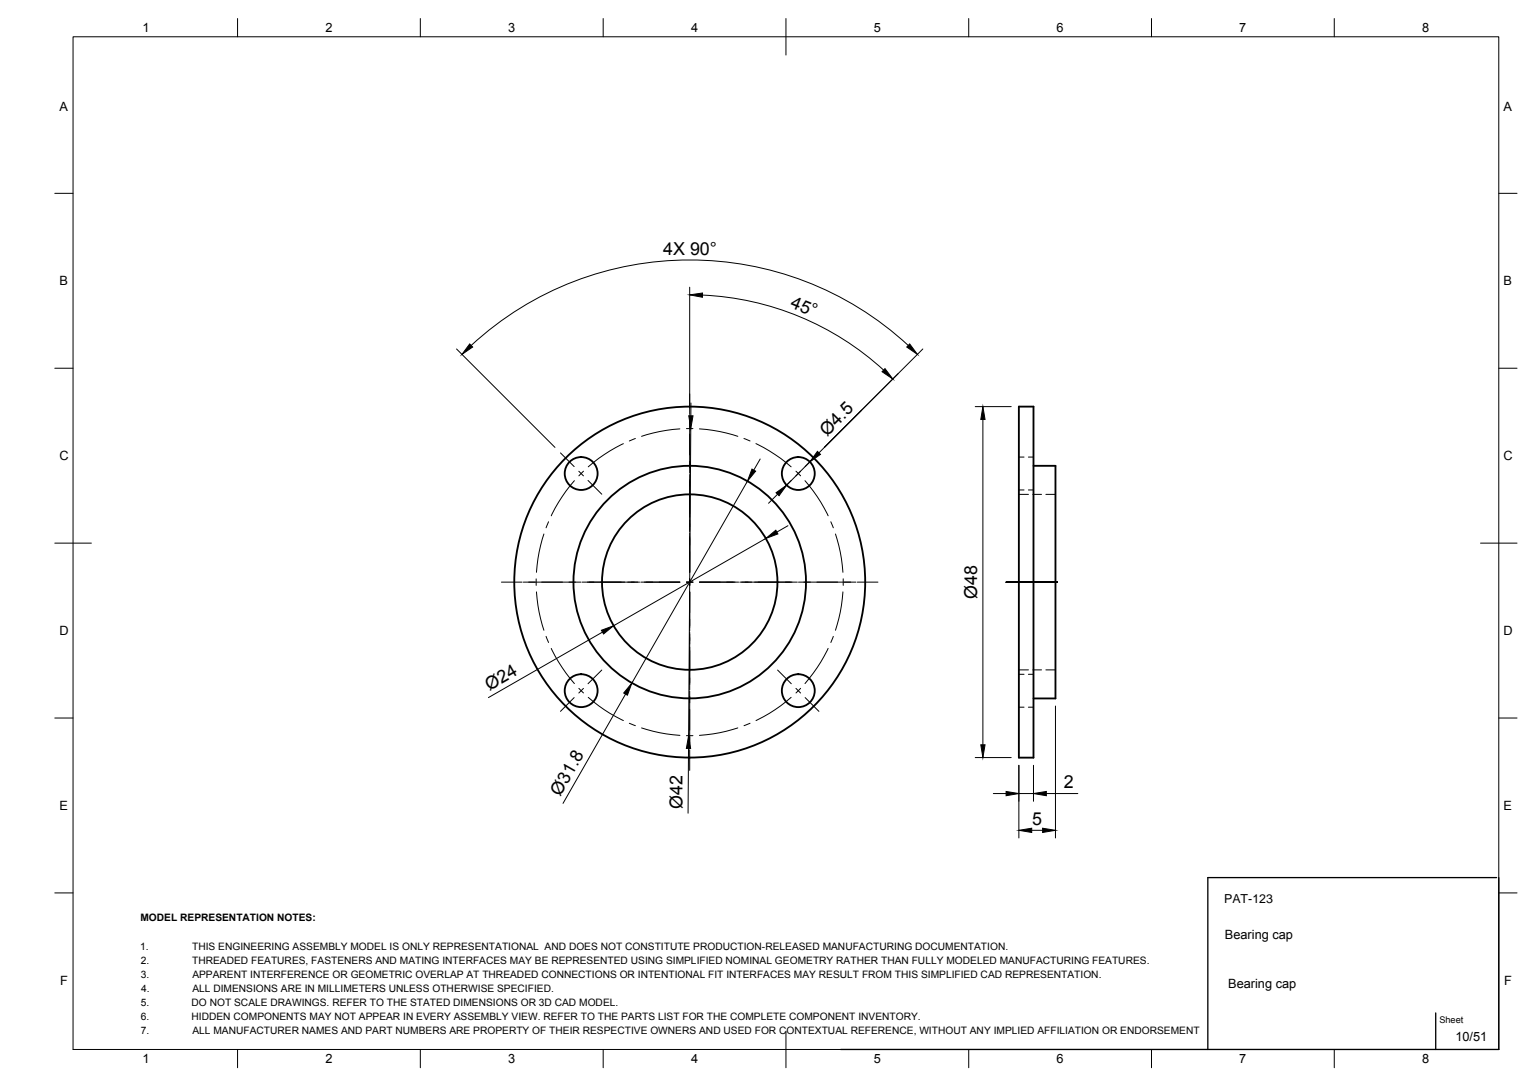
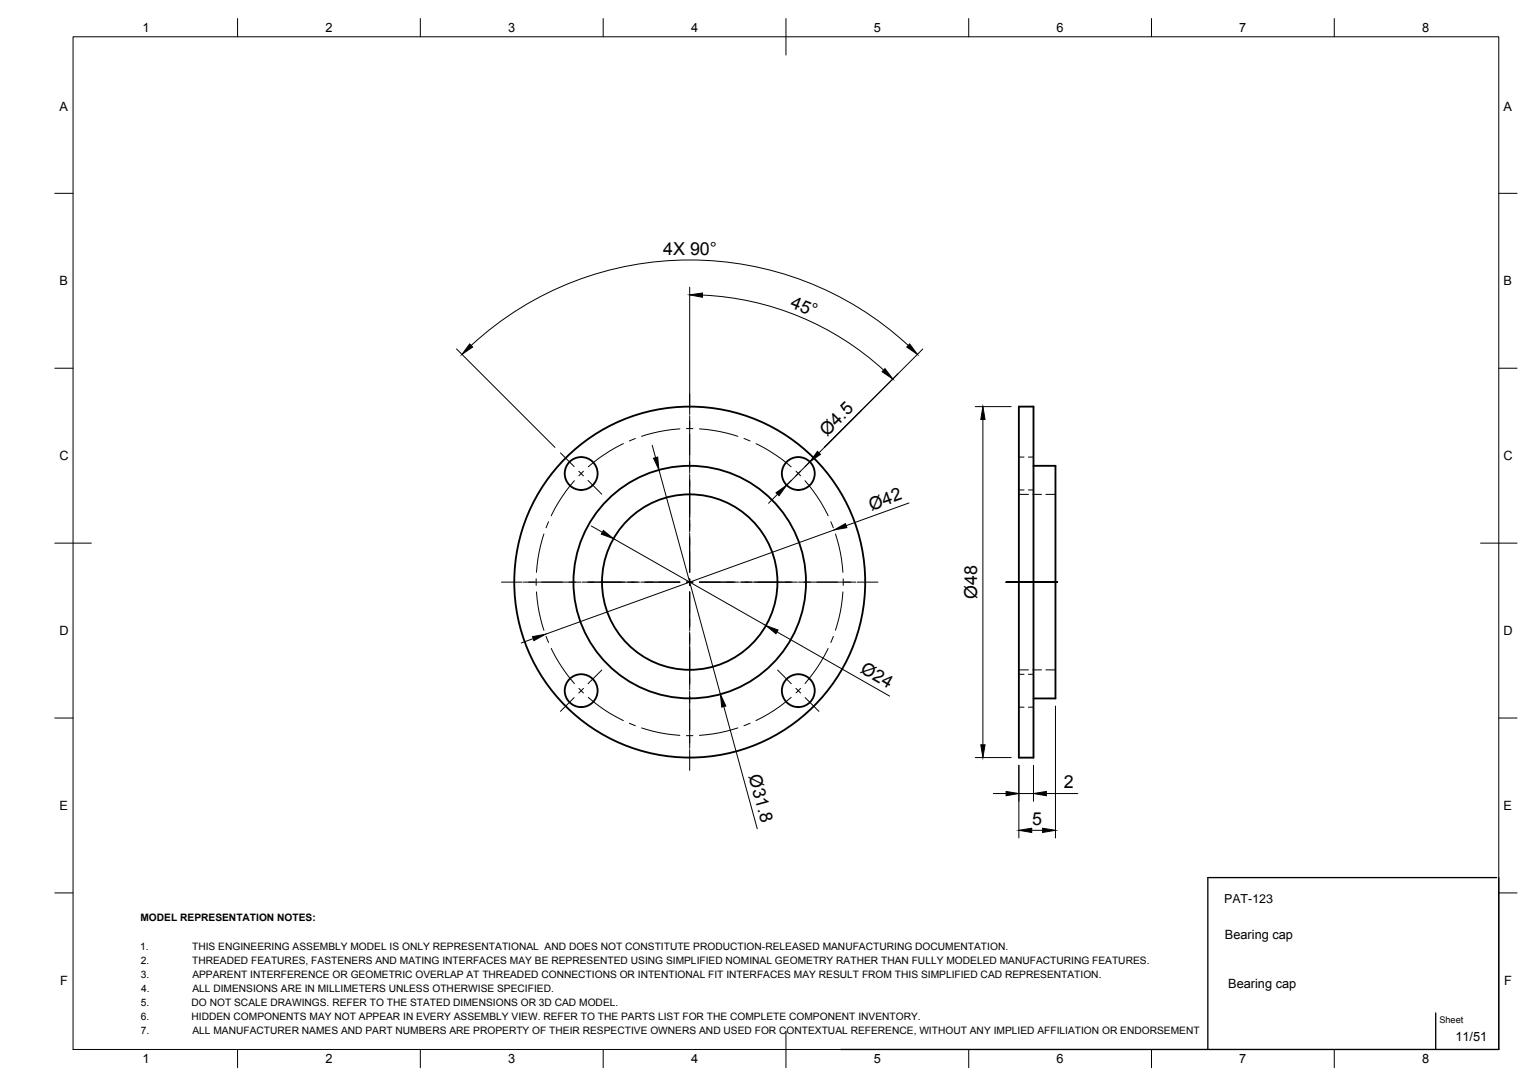
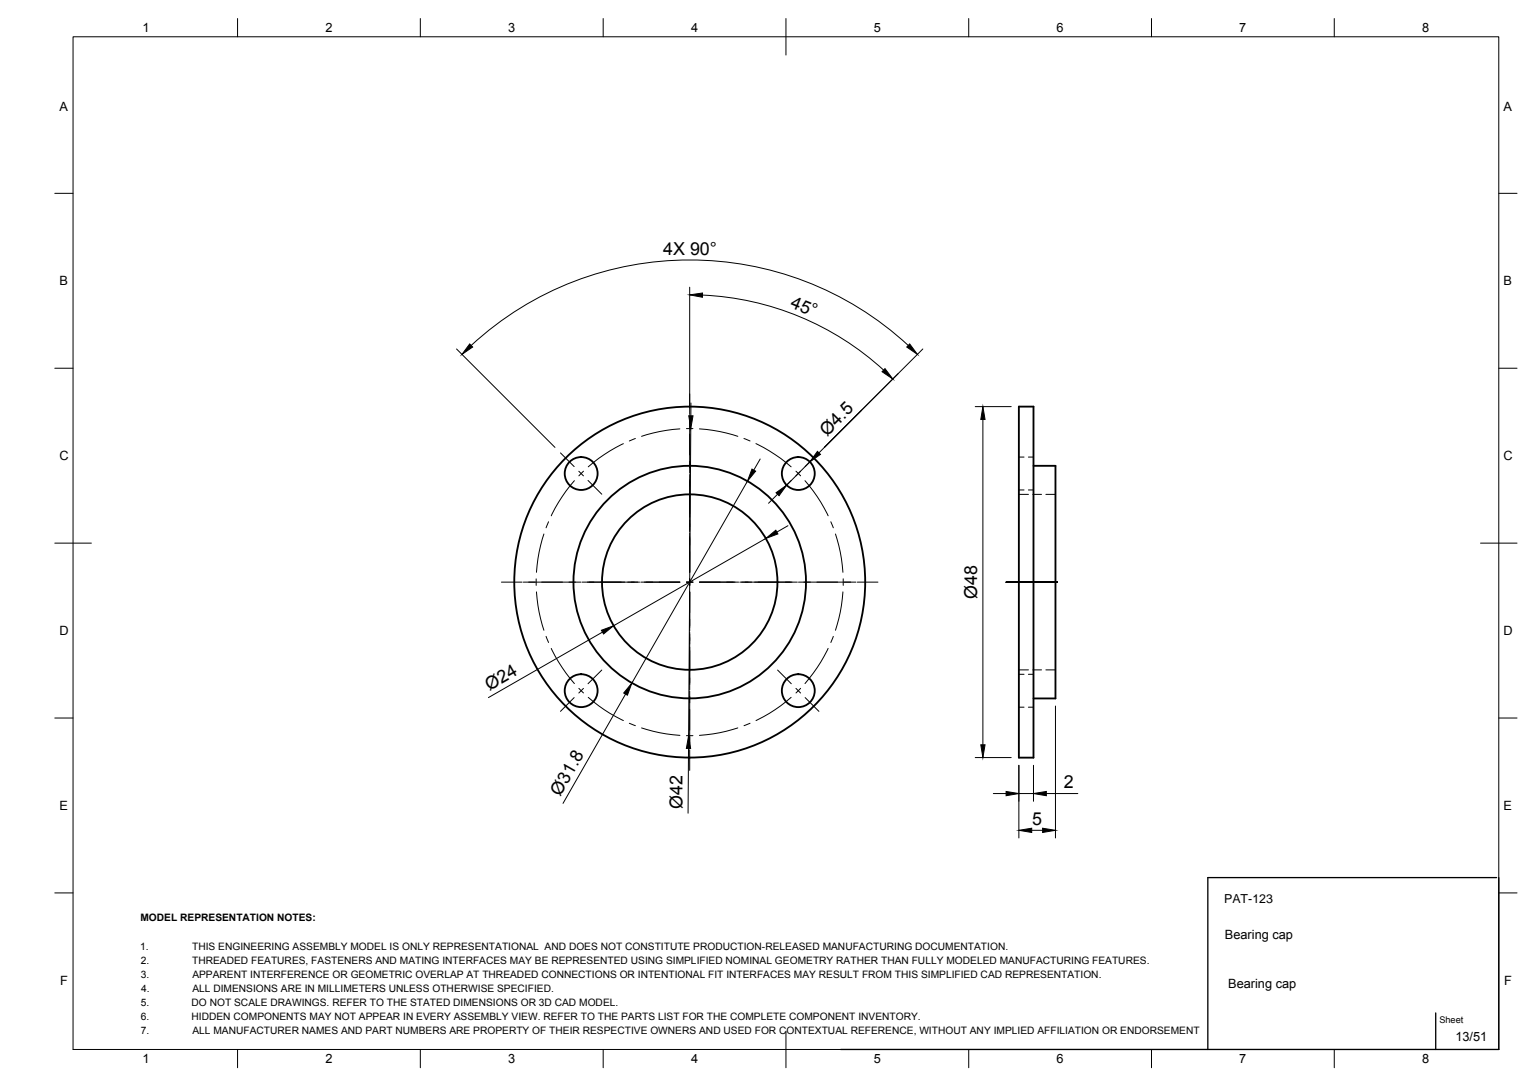
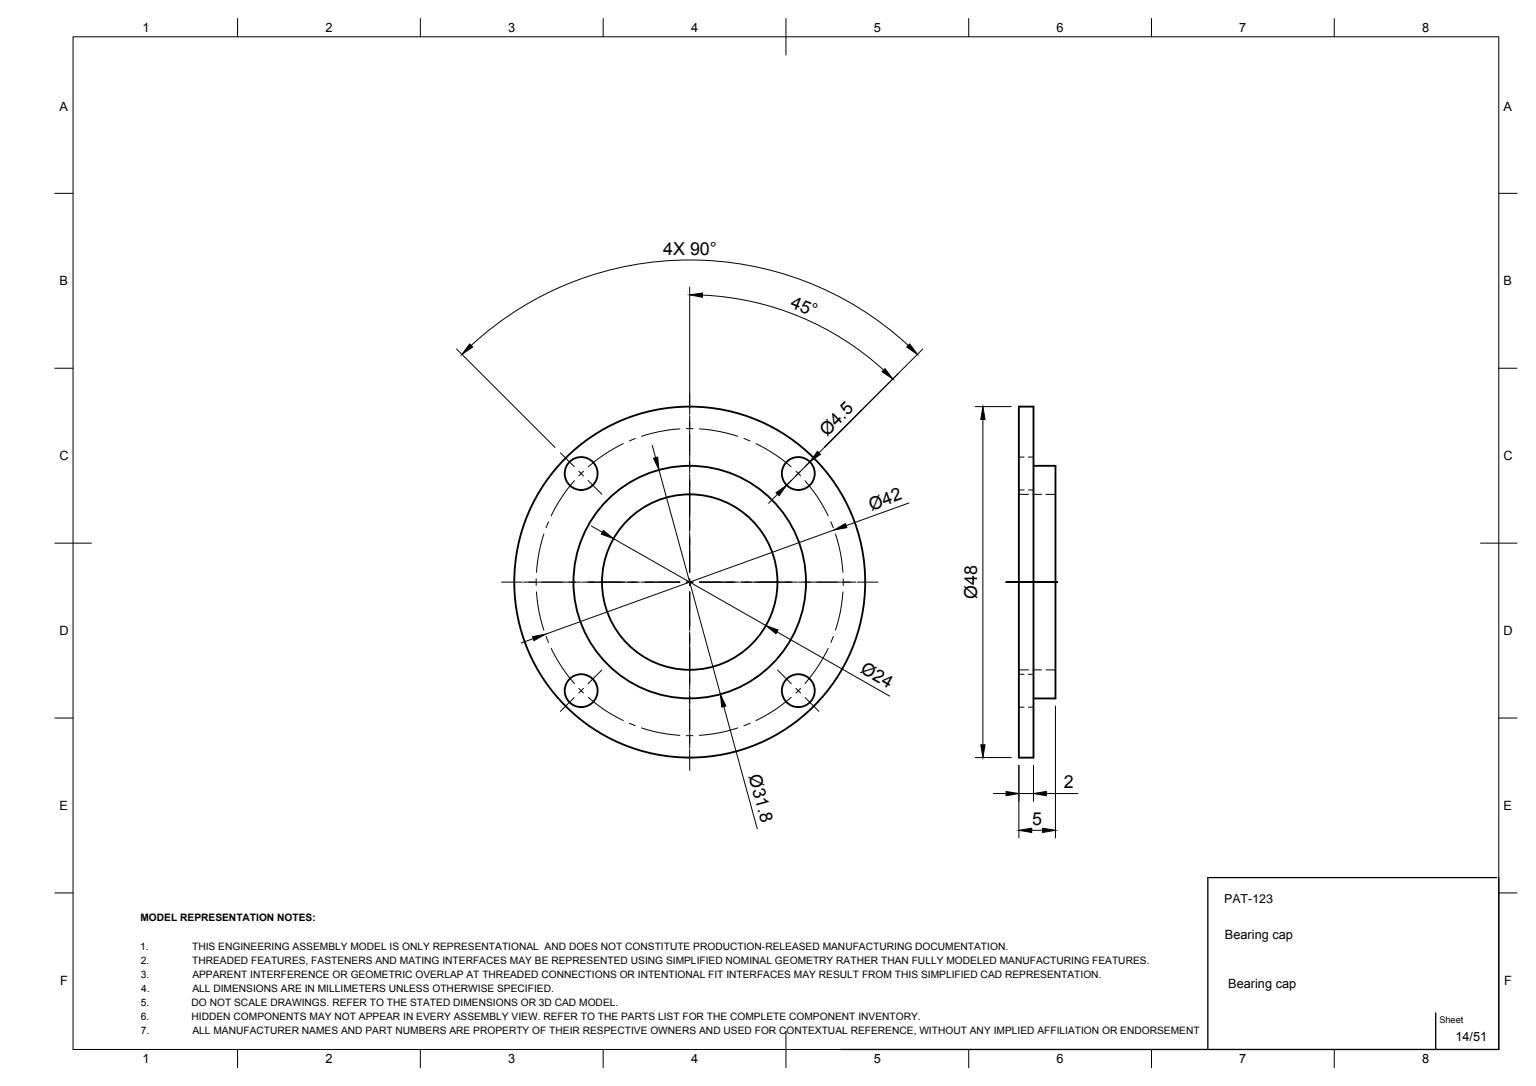
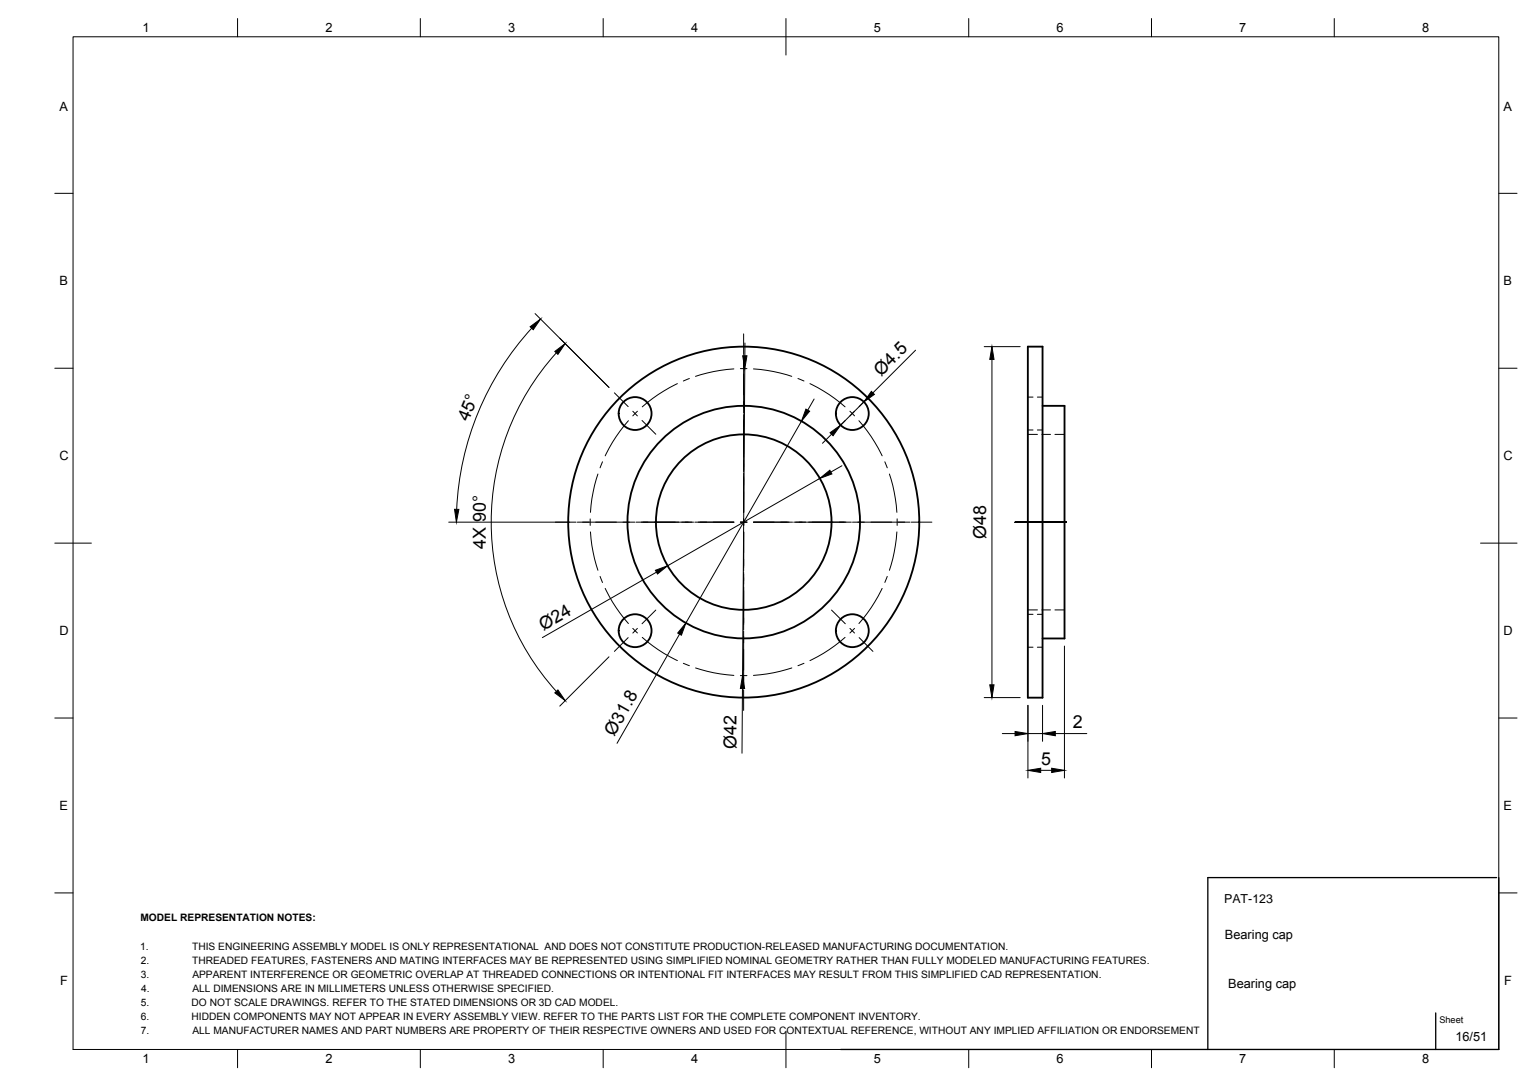
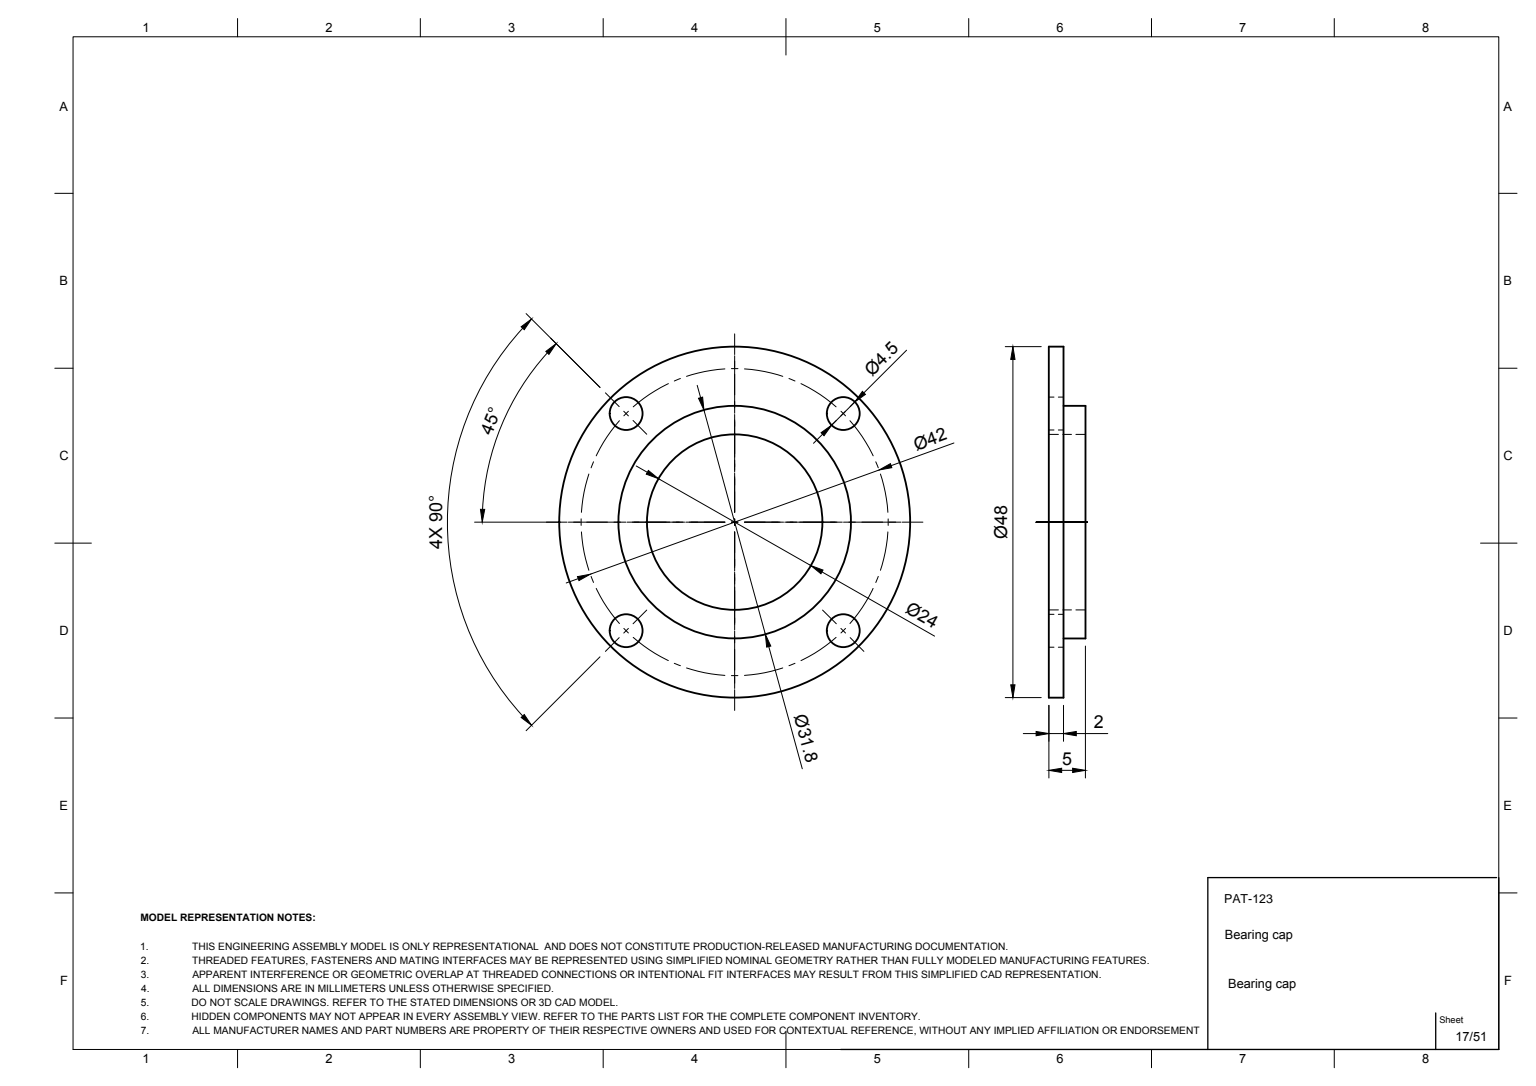
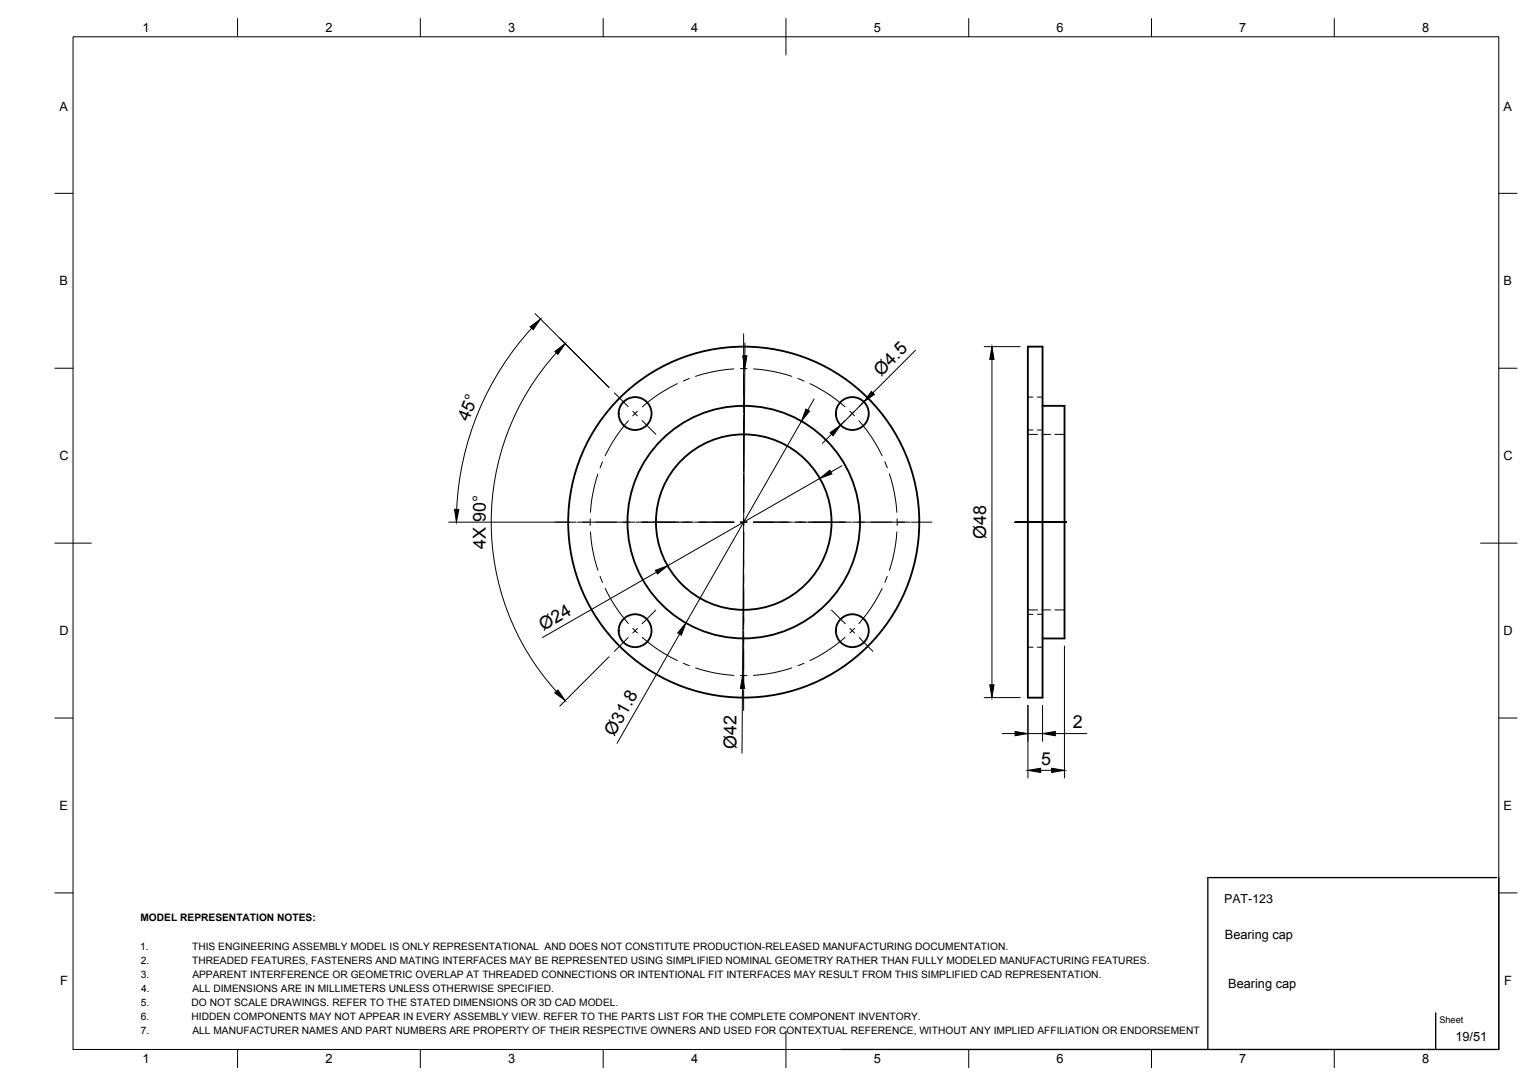
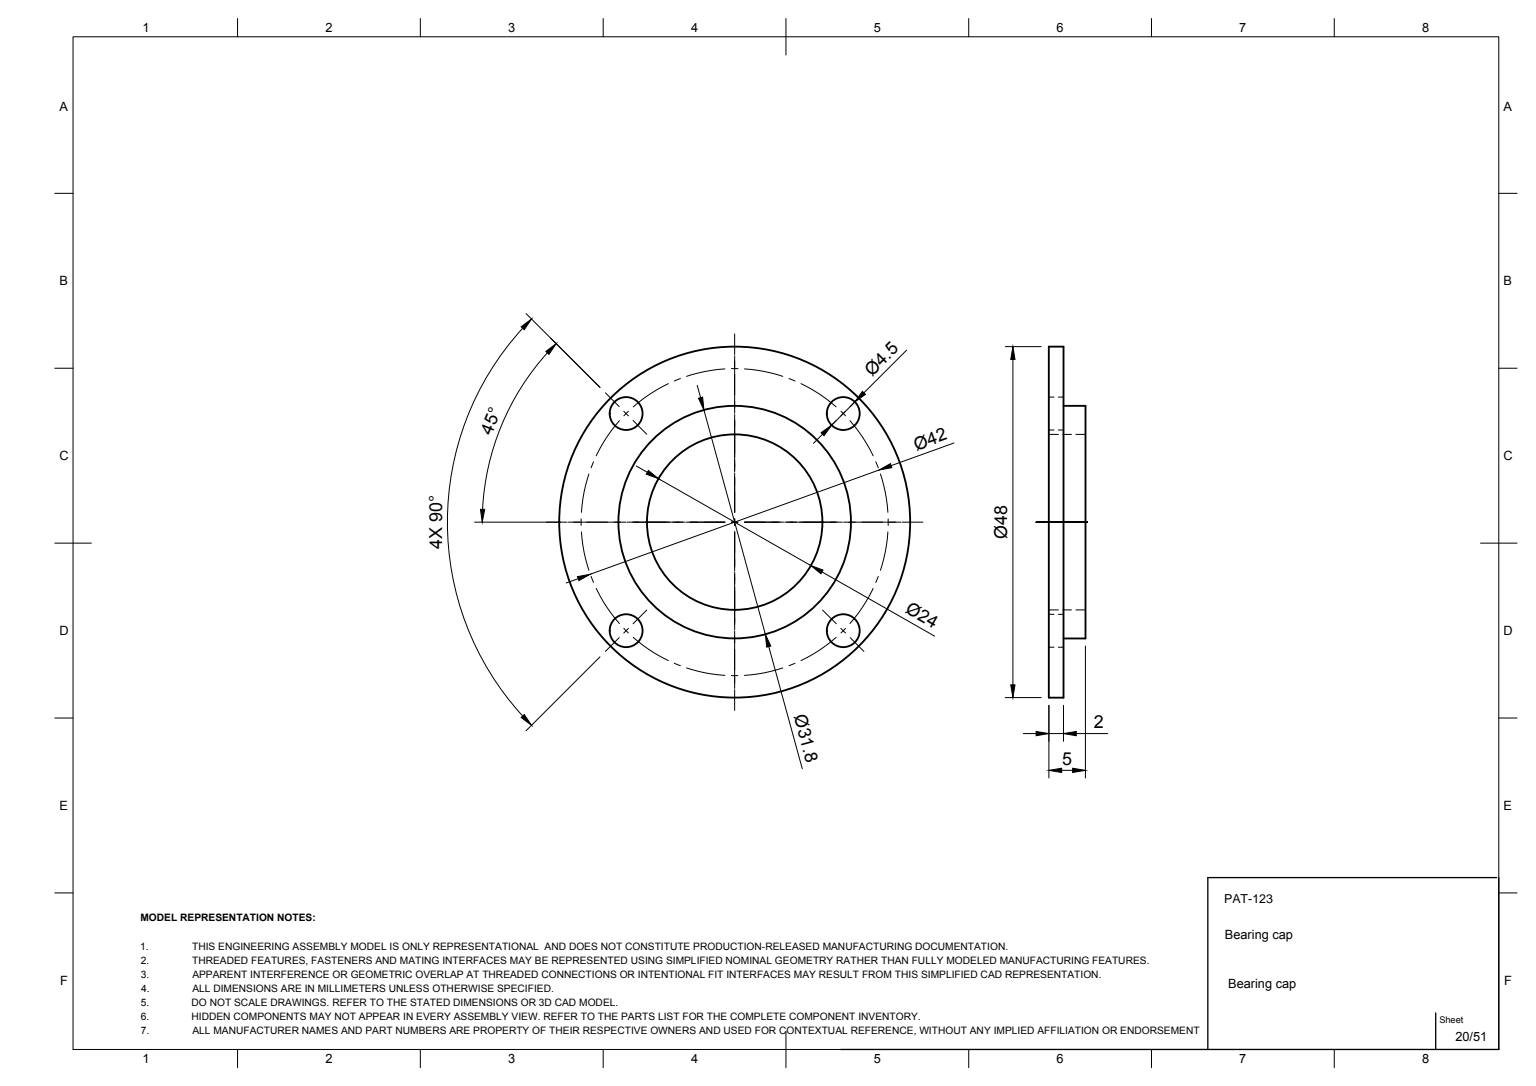
ISO-10303-21;
HEADER;
/* Generated by software containing ST-Developer
 * from STEP Tools, Inc. (www.steptools.com) 
 */

FILE_DESCRIPTION(
/* description */ ('Worm-less right-angle friction wheel drive'),
/* implementation_level */ '2;1');

FILE_NAME(
/* name */ 'Bearing cap.step',
/* time_stamp */ '2026-10-28T03:22:36-07:00',
/* author */ (''),
/* organization */ (''),
/* preprocessor_version */ 'ST-DEVELOPER v20.2',
/* originating_system */ 'Autodesk Translation Framework v15.17.0.0',
/* authorisation */ '');

FILE_SCHEMA (('AUTOMOTIVE_DESIGN { 1 0 10303 214 3 1 1 }'));
ENDSEC;

DATA;
#10=MECHANICAL_DESIGN_GEOMETRIC_PRESENTATION_REPRESENTATION('',(#616),#17046);
#522=SHAPE_REPRESENTATION_RELATIONSHIP('SRR','None',#17265,#569);
#569=ADVANCED_BREP_SHAPE_REPRESENTATION('',(#670),#17001);
#616=STYLED_ITEM('',(#17591),#670);
#670=MANIFOLD_SOLID_BREP('Body1',#8171);
#765=FACE_BOUND('',#1801,.T.);
#766=FACE_BOUND('',#1805,.T.);
#767=FACE_BOUND('',#1806,.T.);
#768=FACE_BOUND('',#1807,.T.);
#769=FACE_BOUND('',#1808,.T.);
#770=FACE_BOUND('',#1809,.T.);
#771=FACE_BOUND('',#1811,.T.);
#772=FACE_BOUND('',#1812,.T.);
#773=FACE_BOUND('',#1813,.T.);
#774=FACE_BOUND('',#1814,.T.);
#775=FACE_BOUND('',#1815,.T.);
#994=PLANE('',#8894);
#995=PLANE('',#8901);
#996=PLANE('',#8902);
#1279=FACE_OUTER_BOUND('',#1795,.T.);
#1280=FACE_OUTER_BOUND('',#1796,.T.);
#1281=FACE_OUTER_BOUND('',#1797,.T.);
#1282=FACE_OUTER_BOUND('',#1798,.T.);
#1283=FACE_OUTER_BOUND('',#1799,.T.);
#1284=FACE_OUTER_BOUND('',#1800,.T.);
#1285=FACE_OUTER_BOUND('',#1802,.T.);
#1286=FACE_OUTER_BOUND('',#1803,.T.);
#1287=FACE_OUTER_BOUND('',#1804,.T.);
#1288=FACE_OUTER_BOUND('',#1810,.T.);
#1795=EDGE_LOOP('',(#5900,#5901,#5902,#5903));
#1796=EDGE_LOOP('',(#5904,#5905,#5906,#5907));
#1797=EDGE_LOOP('',(#5908,#5909,#5910,#5911));
#1798=EDGE_LOOP('',(#5912,#5913,#5914,#5915));
#1799=EDGE_LOOP('',(#5916,#5917,#5918,#5919));
#1800=EDGE_LOOP('',(#5920));
#1801=EDGE_LOOP('',(#5921));
#1802=EDGE_LOOP('',(#5922,#5923,#5924,#5925));
#1803=EDGE_LOOP('',(#5926,#5927,#5928,#5929));
#1804=EDGE_LOOP('',(#5930));
#1805=EDGE_LOOP('',(#5931));
#1806=EDGE_LOOP('',(#5932));
#1807=EDGE_LOOP('',(#5933));
#1808=EDGE_LOOP('',(#5934));
#1809=EDGE_LOOP('',(#5935));
#1810=EDGE_LOOP('',(#5936));
#1811=EDGE_LOOP('',(#5937));
#1812=EDGE_LOOP('',(#5938));
#1813=EDGE_LOOP('',(#5939));
#1814=EDGE_LOOP('',(#5940));
#1815=EDGE_LOOP('',(#5941));
#2502=LINE('',#12763,#3042);
#2503=LINE('',#12769,#3043);
#2504=LINE('',#12775,#3044);
#2505=LINE('',#12781,#3045);
#2506=LINE('',#12787,#3046);
#2507=LINE('',#12794,#3047);
#2508=LINE('',#12800,#3048);
#3042=VECTOR('',#10176,0.225);
#3043=VECTOR('',#10183,0.225);
#3044=VECTOR('',#10190,0.225);
#3045=VECTOR('',#10197,0.225);
#3046=VECTOR('',#10204,1.59);
#3047=VECTOR('',#10213,1.2);
#3048=VECTOR('',#10220,2.4);
#3515=CIRCLE('',#8880,0.225);
#3516=CIRCLE('',#8881,0.225);
#3517=CIRCLE('',#8883,0.225);
#3518=CIRCLE('',#8884,0.225);
#3519=CIRCLE('',#8886,0.225);
#3520=CIRCLE('',#8887,0.225);
#3521=CIRCLE('',#8889,0.225);
#3522=CIRCLE('',#8890,0.225);
#3523=CIRCLE('',#8892,1.59);
#3524=CIRCLE('',#8893,1.59);
#3525=CIRCLE('',#8895,1.2);
#3526=CIRCLE('',#8897,1.2);
#3527=CIRCLE('',#8899,2.4);
#3528=CIRCLE('',#8900,2.4);
#3991=VERTEX_POINT('',#12760);
#3992=VERTEX_POINT('',#12762);
#3993=VERTEX_POINT('',#12766);
#3994=VERTEX_POINT('',#12768);
#3995=VERTEX_POINT('',#12772);
#3996=VERTEX_POINT('',#12774);
#3997=VERTEX_POINT('',#12778);
#3998=VERTEX_POINT('',#12780);
#3999=VERTEX_POINT('',#12784);
#4000=VERTEX_POINT('',#12786);
#4001=VERTEX_POINT('',#12790);
#4002=VERTEX_POINT('',#12793);
#4003=VERTEX_POINT('',#12797);
#4004=VERTEX_POINT('',#12799);
#4719=EDGE_CURVE('',#3991,#3991,#3515,.T.);
#4720=EDGE_CURVE('',#3991,#3992,#2502,.T.);
#4721=EDGE_CURVE('',#3992,#3992,#3516,.T.);
#4722=EDGE_CURVE('',#3993,#3993,#3517,.T.);
#4723=EDGE_CURVE('',#3993,#3994,#2503,.T.);
#4724=EDGE_CURVE('',#3994,#3994,#3518,.T.);
#4725=EDGE_CURVE('',#3995,#3995,#3519,.T.);
#4726=EDGE_CURVE('',#3995,#3996,#2504,.T.);
#4727=EDGE_CURVE('',#3996,#3996,#3520,.T.);
#4728=EDGE_CURVE('',#3997,#3997,#3521,.T.);
#4729=EDGE_CURVE('',#3997,#3998,#2505,.T.);
#4730=EDGE_CURVE('',#3998,#3998,#3522,.T.);
#4731=EDGE_CURVE('',#3999,#3999,#3523,.T.);
#4732=EDGE_CURVE('',#3999,#4000,#2506,.T.);
#4733=EDGE_CURVE('',#4000,#4000,#3524,.T.);
#4734=EDGE_CURVE('',#4001,#4001,#3525,.T.);
#4735=EDGE_CURVE('',#4001,#4002,#2507,.T.);
#4736=EDGE_CURVE('',#4002,#4002,#3526,.T.);
#4737=EDGE_CURVE('',#4003,#4003,#3527,.T.);
#4738=EDGE_CURVE('',#4003,#4004,#2508,.T.);
#4739=EDGE_CURVE('',#4004,#4004,#3528,.T.);
#5900=ORIENTED_EDGE('',*,*,#4719,.F.);
#5901=ORIENTED_EDGE('',*,*,#4720,.T.);
#5902=ORIENTED_EDGE('',*,*,#4721,.F.);
#5903=ORIENTED_EDGE('',*,*,#4720,.F.);
#5904=ORIENTED_EDGE('',*,*,#4722,.F.);
#5905=ORIENTED_EDGE('',*,*,#4723,.T.);
#5906=ORIENTED_EDGE('',*,*,#4724,.F.);
#5907=ORIENTED_EDGE('',*,*,#4723,.F.);
#5908=ORIENTED_EDGE('',*,*,#4725,.F.);
#5909=ORIENTED_EDGE('',*,*,#4726,.T.);
#5910=ORIENTED_EDGE('',*,*,#4727,.F.);
#5911=ORIENTED_EDGE('',*,*,#4726,.F.);
#5912=ORIENTED_EDGE('',*,*,#4728,.F.);
#5913=ORIENTED_EDGE('',*,*,#4729,.T.);
#5914=ORIENTED_EDGE('',*,*,#4730,.F.);
#5915=ORIENTED_EDGE('',*,*,#4729,.F.);
#5916=ORIENTED_EDGE('',*,*,#4731,.F.);
#5917=ORIENTED_EDGE('',*,*,#4732,.T.);
#5918=ORIENTED_EDGE('',*,*,#4733,.F.);
#5919=ORIENTED_EDGE('',*,*,#4732,.F.);
#5920=ORIENTED_EDGE('',*,*,#4731,.T.);
#5921=ORIENTED_EDGE('',*,*,#4734,.T.);
#5922=ORIENTED_EDGE('',*,*,#4734,.F.);
#5923=ORIENTED_EDGE('',*,*,#4735,.T.);
#5924=ORIENTED_EDGE('',*,*,#4736,.T.);
#5925=ORIENTED_EDGE('',*,*,#4735,.F.);
#5926=ORIENTED_EDGE('',*,*,#4737,.F.);
#5927=ORIENTED_EDGE('',*,*,#4738,.T.);
#5928=ORIENTED_EDGE('',*,*,#4739,.T.);
#5929=ORIENTED_EDGE('',*,*,#4738,.F.);
#5930=ORIENTED_EDGE('',*,*,#4737,.T.);
#5931=ORIENTED_EDGE('',*,*,#4733,.T.);
#5932=ORIENTED_EDGE('',*,*,#4730,.T.);
#5933=ORIENTED_EDGE('',*,*,#4727,.T.);
#5934=ORIENTED_EDGE('',*,*,#4724,.T.);
#5935=ORIENTED_EDGE('',*,*,#4721,.T.);
#5936=ORIENTED_EDGE('',*,*,#4739,.F.);
#5937=ORIENTED_EDGE('',*,*,#4736,.F.);
#5938=ORIENTED_EDGE('',*,*,#4728,.T.);
#5939=ORIENTED_EDGE('',*,*,#4725,.T.);
#5940=ORIENTED_EDGE('',*,*,#4722,.T.);
#5941=ORIENTED_EDGE('',*,*,#4719,.T.);
#7559=CYLINDRICAL_SURFACE('',#8879,0.225);
#7560=CYLINDRICAL_SURFACE('',#8882,0.225);
#7561=CYLINDRICAL_SURFACE('',#8885,0.225);
#7562=CYLINDRICAL_SURFACE('',#8888,0.225);
#7563=CYLINDRICAL_SURFACE('',#8891,1.59);
#7564=CYLINDRICAL_SURFACE('',#8896,1.2);
#7565=CYLINDRICAL_SURFACE('',#8898,2.4);
#7771=ADVANCED_FACE('',(#1279),#7559,.F.);
#7772=ADVANCED_FACE('',(#1280),#7560,.F.);
#7773=ADVANCED_FACE('',(#1281),#7561,.F.);
#7774=ADVANCED_FACE('',(#1282),#7562,.F.);
#7775=ADVANCED_FACE('',(#1283),#7563,.T.);
#7776=ADVANCED_FACE('',(#1284,#765),#994,.T.);
#7777=ADVANCED_FACE('',(#1285),#7564,.F.);
#7778=ADVANCED_FACE('',(#1286),#7565,.T.);
#7779=ADVANCED_FACE('',(#1287,#766,#767,#768,#769,#770),#995,.T.);
#7780=ADVANCED_FACE('',(#1288,#771,#772,#773,#774,#775),#996,.F.);
#8171=CLOSED_SHELL('',(#7771,#7772,#7773,#7774,#7775,#7776,#7777,#7778,
#7779,#7780));
#8878=AXIS2_PLACEMENT_3D('',#12758,#10170,#10171);
#8879=AXIS2_PLACEMENT_3D('',#12759,#10172,#10173);
#8880=AXIS2_PLACEMENT_3D('',#12761,#10174,#10175);
#8881=AXIS2_PLACEMENT_3D('',#12764,#10177,#10178);
#8882=AXIS2_PLACEMENT_3D('',#12765,#10179,#10180);
#8883=AXIS2_PLACEMENT_3D('',#12767,#10181,#10182);
#8884=AXIS2_PLACEMENT_3D('',#12770,#10184,#10185);
#8885=AXIS2_PLACEMENT_3D('',#12771,#10186,#10187);
#8886=AXIS2_PLACEMENT_3D('',#12773,#10188,#10189);
#8887=AXIS2_PLACEMENT_3D('',#12776,#10191,#10192);
#8888=AXIS2_PLACEMENT_3D('',#12777,#10193,#10194);
#8889=AXIS2_PLACEMENT_3D('',#12779,#10195,#10196);
#8890=AXIS2_PLACEMENT_3D('',#12782,#10198,#10199);
#8891=AXIS2_PLACEMENT_3D('',#12783,#10200,#10201);
#8892=AXIS2_PLACEMENT_3D('',#12785,#10202,#10203);
#8893=AXIS2_PLACEMENT_3D('',#12788,#10205,#10206);
#8894=AXIS2_PLACEMENT_3D('',#12789,#10207,#10208);
#8895=AXIS2_PLACEMENT_3D('',#12791,#10209,#10210);
#8896=AXIS2_PLACEMENT_3D('',#12792,#10211,#10212);
#8897=AXIS2_PLACEMENT_3D('',#12795,#10214,#10215);
#8898=AXIS2_PLACEMENT_3D('',#12796,#10216,#10217);
#8899=AXIS2_PLACEMENT_3D('',#12798,#10218,#10219);
#8900=AXIS2_PLACEMENT_3D('',#12801,#10221,#10222);
#8901=AXIS2_PLACEMENT_3D('',#12802,#10223,#10224);
#8902=AXIS2_PLACEMENT_3D('',#12803,#10225,#10226);
#10170=DIRECTION('axis',(0.,0.,1.));
#10171=DIRECTION('refdir',(1.,0.,0.));
#10172=DIRECTION('center_axis',(0.,1.,0.));
#10173=DIRECTION('ref_axis',(1.,0.,0.));
#10174=DIRECTION('center_axis',(0.,1.,0.));
#10175=DIRECTION('ref_axis',(1.,0.,0.));
#10176=DIRECTION('',(0.,1.,0.));
#10177=DIRECTION('center_axis',(0.,-1.,0.));
#10178=DIRECTION('ref_axis',(1.,0.,0.));
#10179=DIRECTION('center_axis',(0.,1.,0.));
#10180=DIRECTION('ref_axis',(1.,0.,0.));
#10181=DIRECTION('center_axis',(0.,1.,0.));
#10182=DIRECTION('ref_axis',(1.,0.,0.));
#10183=DIRECTION('',(0.,1.,0.));
#10184=DIRECTION('center_axis',(0.,-1.,0.));
#10185=DIRECTION('ref_axis',(1.,0.,0.));
#10186=DIRECTION('center_axis',(0.,1.,0.));
#10187=DIRECTION('ref_axis',(1.,0.,0.));
#10188=DIRECTION('center_axis',(0.,1.,0.));
#10189=DIRECTION('ref_axis',(1.,0.,0.));
#10190=DIRECTION('',(0.,1.,0.));
#10191=DIRECTION('center_axis',(0.,-1.,0.));
#10192=DIRECTION('ref_axis',(1.,0.,0.));
#10193=DIRECTION('center_axis',(0.,1.,0.));
#10194=DIRECTION('ref_axis',(1.,0.,0.));
#10195=DIRECTION('center_axis',(0.,1.,0.));
#10196=DIRECTION('ref_axis',(1.,0.,0.));
#10197=DIRECTION('',(0.,1.,0.));
#10198=DIRECTION('center_axis',(0.,-1.,0.));
#10199=DIRECTION('ref_axis',(1.,0.,0.));
#10200=DIRECTION('center_axis',(0.,1.,0.));
#10201=DIRECTION('ref_axis',(1.,0.,0.));
#10202=DIRECTION('center_axis',(0.,1.,0.));
#10203=DIRECTION('ref_axis',(1.,0.,0.));
#10204=DIRECTION('',(0.,-1.,0.));
#10205=DIRECTION('center_axis',(0.,-1.,0.));
#10206=DIRECTION('ref_axis',(1.,0.,0.));
#10207=DIRECTION('center_axis',(0.,1.,0.));
#10208=DIRECTION('ref_axis',(1.,0.,0.));
#10209=DIRECTION('center_axis',(0.,-1.,0.));
#10210=DIRECTION('ref_axis',(1.,0.,0.));
#10211=DIRECTION('center_axis',(0.,1.,0.));
#10212=DIRECTION('ref_axis',(1.,0.,0.));
#10213=DIRECTION('',(0.,-1.,0.));
#10214=DIRECTION('center_axis',(0.,-1.,0.));
#10215=DIRECTION('ref_axis',(1.,0.,0.));
#10216=DIRECTION('center_axis',(0.,1.,0.));
#10217=DIRECTION('ref_axis',(1.,0.,0.));
#10218=DIRECTION('center_axis',(0.,1.,0.));
#10219=DIRECTION('ref_axis',(1.,0.,0.));
#10220=DIRECTION('',(0.,-1.,0.));
#10221=DIRECTION('center_axis',(0.,1.,0.));
#10222=DIRECTION('ref_axis',(1.,0.,0.));
#10223=DIRECTION('center_axis',(0.,1.,0.));
#10224=DIRECTION('ref_axis',(1.,0.,0.));
#10225=DIRECTION('center_axis',(0.,1.,0.));
#10226=DIRECTION('ref_axis',(1.,0.,0.));
#12758=CARTESIAN_POINT('',(0.,0.,0.));
#12759=CARTESIAN_POINT('Origin',(-1.48492424049175,-8.1,5.51507575950825));
#12760=CARTESIAN_POINT('',(-1.70992424049175,-8.,5.51507575950825));
#12761=CARTESIAN_POINT('Origin',(-1.48492424049175,-8.,5.51507575950825));
#12762=CARTESIAN_POINT('',(-1.70992424049175,-7.8,5.51507575950825));
#12763=CARTESIAN_POINT('',(-1.70992424049175,-8.1,5.51507575950825));
#12764=CARTESIAN_POINT('Origin',(-1.48492424049175,-7.8,5.51507575950825));
#12765=CARTESIAN_POINT('Origin',(-1.48492424049175,-8.1,8.48492424049175));
#12766=CARTESIAN_POINT('',(-1.70992424049175,-8.,8.48492424049175));
#12767=CARTESIAN_POINT('Origin',(-1.48492424049175,-8.,8.48492424049175));
#12768=CARTESIAN_POINT('',(-1.70992424049175,-7.8,8.48492424049175));
#12769=CARTESIAN_POINT('',(-1.70992424049175,-8.1,8.48492424049175));
#12770=CARTESIAN_POINT('Origin',(-1.48492424049175,-7.8,8.48492424049175));
#12771=CARTESIAN_POINT('Origin',(1.48492424049175,-8.1,8.48492424049175));
#12772=CARTESIAN_POINT('',(1.25992424049175,-8.,8.48492424049175));
#12773=CARTESIAN_POINT('Origin',(1.48492424049175,-8.,8.48492424049175));
#12774=CARTESIAN_POINT('',(1.25992424049175,-7.8,8.48492424049175));
#12775=CARTESIAN_POINT('',(1.25992424049175,-8.1,8.48492424049175));
#12776=CARTESIAN_POINT('Origin',(1.48492424049175,-7.8,8.48492424049175));
#12777=CARTESIAN_POINT('Origin',(1.48492424049175,-8.1,5.51507575950825));
#12778=CARTESIAN_POINT('',(1.25992424049175,-8.,5.51507575950825));
#12779=CARTESIAN_POINT('Origin',(1.48492424049175,-8.,5.51507575950825));
#12780=CARTESIAN_POINT('',(1.25992424049175,-7.8,5.51507575950825));
#12781=CARTESIAN_POINT('',(1.25992424049175,-8.1,5.51507575950825));
#12782=CARTESIAN_POINT('Origin',(1.48492424049175,-7.8,5.51507575950825));
#12783=CARTESIAN_POINT('Origin',(0.,-7.8,7.));
#12784=CARTESIAN_POINT('',(-1.59,-7.5,7.));
#12785=CARTESIAN_POINT('Origin',(0.,-7.5,7.));
#12786=CARTESIAN_POINT('',(-1.59,-7.8,7.));
#12787=CARTESIAN_POINT('',(-1.59,-7.8,7.));
#12788=CARTESIAN_POINT('Origin',(0.,-7.8,7.));
#12789=CARTESIAN_POINT('Origin',(0.,-7.5,7.));
#12790=CARTESIAN_POINT('',(-1.2,-7.5,7.));
#12791=CARTESIAN_POINT('Origin',(0.,-7.5,7.));
#12792=CARTESIAN_POINT('Origin',(0.,-8.,7.));
#12793=CARTESIAN_POINT('',(-1.2,-8.,7.));
#12794=CARTESIAN_POINT('',(-1.2,-8.,7.));
#12795=CARTESIAN_POINT('Origin',(0.,-8.,7.));
#12796=CARTESIAN_POINT('Origin',(0.,-8.,7.));
#12797=CARTESIAN_POINT('',(-2.4,-7.8,7.));
#12798=CARTESIAN_POINT('Origin',(0.,-7.8,7.));
#12799=CARTESIAN_POINT('',(-2.4,-8.,7.));
#12800=CARTESIAN_POINT('',(-2.4,-8.,7.));
#12801=CARTESIAN_POINT('Origin',(0.,-8.,7.));
#12802=CARTESIAN_POINT('Origin',(0.,-7.8,7.));
#12803=CARTESIAN_POINT('Origin',(0.,-8.,7.));
#16948=UNCERTAINTY_MEASURE_WITH_UNIT(LENGTH_MEASURE(0.001),#17047,
'DISTANCE_ACCURACY_VALUE',
'Maximum model space distance between geometric entities at asserted c
onnectivities');
#16993=UNCERTAINTY_MEASURE_WITH_UNIT(LENGTH_MEASURE(0.001),#17047,
'DISTANCE_ACCURACY_VALUE',
'Maximum model space distance between geometric entities at asserted c
onnectivities');
#17001=(
GEOMETRIC_REPRESENTATION_CONTEXT(3)
GLOBAL_UNCERTAINTY_ASSIGNED_CONTEXT((#16948))
GLOBAL_UNIT_ASSIGNED_CONTEXT((#17047,#17049,#17050))
REPRESENTATION_CONTEXT('','3D')
);
#17046=(
GEOMETRIC_REPRESENTATION_CONTEXT(3)
GLOBAL_UNCERTAINTY_ASSIGNED_CONTEXT((#16993))
GLOBAL_UNIT_ASSIGNED_CONTEXT((#17047,#17049,#17050))
REPRESENTATION_CONTEXT('','3D')
);
#17047=(
LENGTH_UNIT()
NAMED_UNIT(*)
SI_UNIT(.CENTI.,.METRE.)
);
#17049=(
NAMED_UNIT(*)
PLANE_ANGLE_UNIT()
SI_UNIT($,.RADIAN.)
);
#17050=(
NAMED_UNIT(*)
SI_UNIT($,.STERADIAN.)
SOLID_ANGLE_UNIT()
);
#17058=SHAPE_DEFINITION_REPRESENTATION(#17110,#17265);
#17110=PRODUCT_DEFINITION_SHAPE('',$,#17318);
#17265=SHAPE_REPRESENTATION('',(#8878),#17001);
#17310=PRODUCT_DEFINITION_CONTEXT('part definition',#17468,'design');
#17318=PRODUCT_DEFINITION('Bearing cap','Bearing cap',#17370,#17310);
#17370=PRODUCT_DEFINITION_FORMATION('',$,#17477);
#17468=APPLICATION_CONTEXT(
'Core Data for Automotive Mechanical Design Process');
#17469=PRODUCT_CONTEXT('part definition',#17468,'mechanical');
#17477=PRODUCT('Bearing cap','Bearing cap','Bearing cap',(#17469));
#17585=COLOUR_RGB('Grey',0.48,0.52,0.57);
#17586=FILL_AREA_STYLE_COLOUR('',#17585);
#17587=FILL_AREA_STYLE('',(#17586));
#17588=SURFACE_STYLE_FILL_AREA(#17587);
#17589=SURFACE_SIDE_STYLE('',(#17588));
#17590=SURFACE_STYLE_USAGE(.BOTH.,#17589);
#17591=PRESENTATION_STYLE_ASSIGNMENT((#17590));
ENDSEC;
END-ISO-10303-21;
